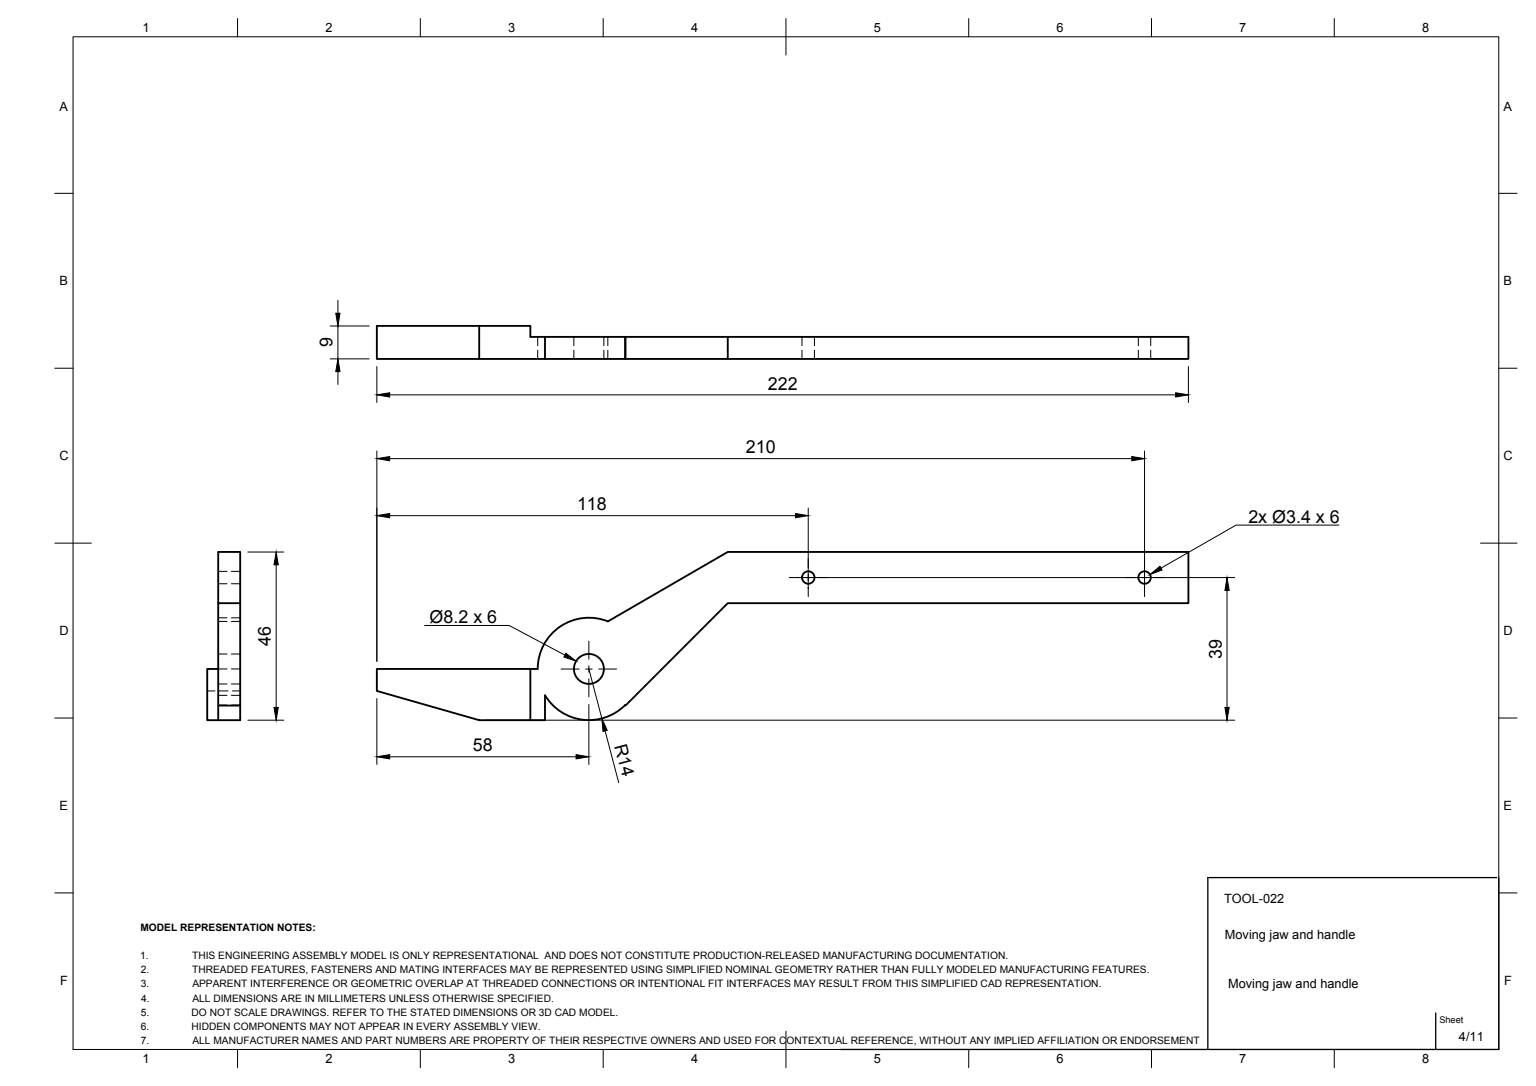
ISO-10303-21;
HEADER;
/* Generated by software containing ST-Developer
 * from STEP Tools, Inc. (www.steptools.com) 
 */

FILE_DESCRIPTION(
/* description */ (''),
/* implementation_level */ '2;1');

FILE_NAME(
/* name */ 'Moving jaw and handle.step',
/* time_stamp */ '2026-11-10T08:27:36-08:00',
/* author */ (''),
/* organization */ (''),
/* preprocessor_version */ 'ST-DEVELOPER v20.2',
/* originating_system */ 'Autodesk Translation Framework v15.17.0.0',
/* authorisation */ '');

FILE_SCHEMA (('AUTOMOTIVE_DESIGN { 1 0 10303 214 3 1 1 }'));
ENDSEC;

DATA;
#10=MECHANICAL_DESIGN_GEOMETRIC_PRESENTATION_REPRESENTATION('',(#567),#19090);
#547=SHAPE_REPRESENTATION_RELATIONSHIP('SRR','None',#19137,#557);
#557=ADVANCED_BREP_SHAPE_REPRESENTATION('',(#577),#19080);
#567=STYLED_ITEM('',(#19200),#577);
#577=MANIFOLD_SOLID_BREP('Body1',#6821);
#592=FACE_BOUND('',#1245,.T.);
#593=FACE_BOUND('',#1246,.T.);
#594=FACE_BOUND('',#1247,.T.);
#595=FACE_BOUND('',#1256,.T.);
#596=FACE_BOUND('',#1257,.T.);
#597=FACE_BOUND('',#1258,.T.);
#675=PLANE('',#6990);
#676=PLANE('',#6991);
#677=PLANE('',#6992);
#678=PLANE('',#6993);
#679=PLANE('',#6994);
#680=PLANE('',#6995);
#681=PLANE('',#6996);
#682=PLANE('',#6997);
#683=PLANE('',#7002);
#684=PLANE('',#7003);
#685=PLANE('',#7004);
#686=PLANE('',#7005);
#687=PLANE('',#7006);
#688=PLANE('',#7007);
#689=PLANE('',#7008);
#840=FACE_OUTER_BOUND('',#1234,.T.);
#841=FACE_OUTER_BOUND('',#1235,.T.);
#842=FACE_OUTER_BOUND('',#1236,.T.);
#843=FACE_OUTER_BOUND('',#1237,.T.);
#844=FACE_OUTER_BOUND('',#1238,.T.);
#845=FACE_OUTER_BOUND('',#1239,.T.);
#846=FACE_OUTER_BOUND('',#1240,.T.);
#847=FACE_OUTER_BOUND('',#1241,.T.);
#848=FACE_OUTER_BOUND('',#1242,.T.);
#849=FACE_OUTER_BOUND('',#1243,.T.);
#850=FACE_OUTER_BOUND('',#1244,.T.);
#851=FACE_OUTER_BOUND('',#1248,.T.);
#852=FACE_OUTER_BOUND('',#1249,.T.);
#853=FACE_OUTER_BOUND('',#1250,.T.);
#854=FACE_OUTER_BOUND('',#1251,.T.);
#855=FACE_OUTER_BOUND('',#1252,.T.);
#856=FACE_OUTER_BOUND('',#1253,.T.);
#857=FACE_OUTER_BOUND('',#1254,.T.);
#858=FACE_OUTER_BOUND('',#1255,.T.);
#859=FACE_OUTER_BOUND('',#1259,.T.);
#1234=EDGE_LOOP('',(#4477,#4478,#4479,#4480));
#1235=EDGE_LOOP('',(#4481,#4482,#4483,#4484));
#1236=EDGE_LOOP('',(#4485,#4486,#4487,#4488));
#1237=EDGE_LOOP('',(#4489,#4490,#4491,#4492));
#1238=EDGE_LOOP('',(#4493,#4494,#4495,#4496,#4497));
#1239=EDGE_LOOP('',(#4498,#4499,#4500,#4501,#4502,#4503));
#1240=EDGE_LOOP('',(#4504,#4505,#4506,#4507));
#1241=EDGE_LOOP('',(#4508,#4509,#4510,#4511));
#1242=EDGE_LOOP('',(#4512,#4513,#4514,#4515));
#1243=EDGE_LOOP('',(#4516,#4517,#4518,#4519,#4520,#4521));
#1244=EDGE_LOOP('',(#4522,#4523,#4524,#4525,#4526,#4527,#4528,#4529,#4530,
#4531,#4532,#4533));
#1245=EDGE_LOOP('',(#4534));
#1246=EDGE_LOOP('',(#4535));
#1247=EDGE_LOOP('',(#4536));
#1248=EDGE_LOOP('',(#4537,#4538,#4539,#4540));
#1249=EDGE_LOOP('',(#4541,#4542,#4543,#4544));
#1250=EDGE_LOOP('',(#4545,#4546,#4547,#4548));
#1251=EDGE_LOOP('',(#4549,#4550,#4551,#4552));
#1252=EDGE_LOOP('',(#4553,#4554,#4555,#4556));
#1253=EDGE_LOOP('',(#4557,#4558,#4559,#4560));
#1254=EDGE_LOOP('',(#4561,#4562,#4563,#4564));
#1255=EDGE_LOOP('',(#4565,#4566,#4567,#4568,#4569,#4570,#4571,#4572,#4573,
#4574,#4575,#4576,#4577));
#1256=EDGE_LOOP('',(#4578));
#1257=EDGE_LOOP('',(#4579));
#1258=EDGE_LOOP('',(#4580));
#1259=EDGE_LOOP('',(#4581,#4582,#4583,#4584));
#1717=LINE('',#9029,#2166);
#1718=LINE('',#9035,#2167);
#1719=LINE('',#9041,#2168);
#1720=LINE('',#9046,#2169);
#1721=LINE('',#9048,#2170);
#1722=LINE('',#9050,#2171);
#1723=LINE('',#9051,#2172);
#1724=LINE('',#9054,#2173);
#1725=LINE('',#9056,#2174);
#1726=LINE('',#9058,#2175);
#1727=LINE('',#9059,#2176);
#1728=LINE('',#9063,#2177);
#1729=LINE('',#9065,#2178);
#1730=LINE('',#9066,#2179);
#1731=LINE('',#9067,#2180);
#1732=LINE('',#9071,#2181);
#1733=LINE('',#9073,#2182);
#1734=LINE('',#9075,#2183);
#1735=LINE('',#9076,#2184);
#1736=LINE('',#9079,#2185);
#1737=LINE('',#9080,#2186);
#1738=LINE('',#9083,#2187);
#1739=LINE('',#9084,#2188);
#1740=LINE('',#9086,#2189);
#1741=LINE('',#9087,#2190);
#1742=LINE('',#9092,#2191);
#1743=LINE('',#9094,#2192);
#1744=LINE('',#9096,#2193);
#1745=LINE('',#9098,#2194);
#1746=LINE('',#9100,#2195);
#1747=LINE('',#9102,#2196);
#1748=LINE('',#9107,#2197);
#1749=LINE('',#9110,#2198);
#1750=LINE('',#9112,#2199);
#1751=LINE('',#9113,#2200);
#1752=LINE('',#9116,#2201);
#1753=LINE('',#9117,#2202);
#1754=LINE('',#9120,#2203);
#1755=LINE('',#9121,#2204);
#1756=LINE('',#9124,#2205);
#1757=LINE('',#9125,#2206);
#1758=LINE('',#9128,#2207);
#1759=LINE('',#9129,#2208);
#1760=LINE('',#9131,#2209);
#2166=VECTOR('',#7582,0.17);
#2167=VECTOR('',#7589,0.17);
#2168=VECTOR('',#7596,0.41);
#2169=VECTOR('',#7601,1.);
#2170=VECTOR('',#7602,1.);
#2171=VECTOR('',#7603,1.);
#2172=VECTOR('',#7604,1.);
#2173=VECTOR('',#7607,1.);
#2174=VECTOR('',#7608,1.);
#2175=VECTOR('',#7609,1.);
#2176=VECTOR('',#7610,1.);
#2177=VECTOR('',#7613,1.);
#2178=VECTOR('',#7614,1.);
#2179=VECTOR('',#7615,1.);
#2180=VECTOR('',#7616,1.);
#2181=VECTOR('',#7619,1.);
#2182=VECTOR('',#7620,1.);
#2183=VECTOR('',#7621,1.);
#2184=VECTOR('',#7622,1.);
#2185=VECTOR('',#7625,1.);
#2186=VECTOR('',#7626,1.);
#2187=VECTOR('',#7629,1.);
#2188=VECTOR('',#7630,1.);
#2189=VECTOR('',#7633,1.);
#2190=VECTOR('',#7634,1.);
#2191=VECTOR('',#7639,1.);
#2192=VECTOR('',#7640,1.);
#2193=VECTOR('',#7641,1.);
#2194=VECTOR('',#7642,1.);
#2195=VECTOR('',#7643,1.);
#2196=VECTOR('',#7644,1.);
#2197=VECTOR('',#7651,1.);
#2198=VECTOR('',#7654,1.);
#2199=VECTOR('',#7655,1.);
#2200=VECTOR('',#7656,1.);
#2201=VECTOR('',#7659,1.);
#2202=VECTOR('',#7660,1.);
#2203=VECTOR('',#7663,1.);
#2204=VECTOR('',#7664,1.);
#2205=VECTOR('',#7667,1.);
#2206=VECTOR('',#7668,1.);
#2207=VECTOR('',#7671,1.);
#2208=VECTOR('',#7672,1.);
#2209=VECTOR('',#7675,1.);
#2564=CIRCLE('',#6982,0.17);
#2565=CIRCLE('',#6983,0.17);
#2566=CIRCLE('',#6985,0.17);
#2567=CIRCLE('',#6986,0.17);
#2568=CIRCLE('',#6988,0.41);
#2569=CIRCLE('',#6989,0.41);
#2570=CIRCLE('',#6998,1.4);
#2571=CIRCLE('',#6999,1.4);
#2572=CIRCLE('',#7001,1.4);
#2573=CIRCLE('',#7009,1.4);
#2760=VERTEX_POINT('',#9026);
#2761=VERTEX_POINT('',#9028);
#2762=VERTEX_POINT('',#9032);
#2763=VERTEX_POINT('',#9034);
#2764=VERTEX_POINT('',#9038);
#2765=VERTEX_POINT('',#9040);
#2766=VERTEX_POINT('',#9044);
#2767=VERTEX_POINT('',#9045);
#2768=VERTEX_POINT('',#9047);
#2769=VERTEX_POINT('',#9049);
#2770=VERTEX_POINT('',#9053);
#2771=VERTEX_POINT('',#9055);
#2772=VERTEX_POINT('',#9057);
#2773=VERTEX_POINT('',#9061);
#2774=VERTEX_POINT('',#9062);
#2775=VERTEX_POINT('',#9064);
#2776=VERTEX_POINT('',#9069);
#2777=VERTEX_POINT('',#9070);
#2778=VERTEX_POINT('',#9072);
#2779=VERTEX_POINT('',#9074);
#2780=VERTEX_POINT('',#9078);
#2781=VERTEX_POINT('',#9082);
#2782=VERTEX_POINT('',#9089);
#2783=VERTEX_POINT('',#9091);
#2784=VERTEX_POINT('',#9093);
#2785=VERTEX_POINT('',#9095);
#2786=VERTEX_POINT('',#9097);
#2787=VERTEX_POINT('',#9099);
#2788=VERTEX_POINT('',#9101);
#2789=VERTEX_POINT('',#9105);
#2790=VERTEX_POINT('',#9109);
#2791=VERTEX_POINT('',#9111);
#2792=VERTEX_POINT('',#9115);
#2793=VERTEX_POINT('',#9119);
#2794=VERTEX_POINT('',#9123);
#2795=VERTEX_POINT('',#9127);
#3423=EDGE_CURVE('',#2760,#2760,#2564,.T.);
#3424=EDGE_CURVE('',#2760,#2761,#1717,.T.);
#3425=EDGE_CURVE('',#2761,#2761,#2565,.T.);
#3426=EDGE_CURVE('',#2762,#2762,#2566,.T.);
#3427=EDGE_CURVE('',#2762,#2763,#1718,.T.);
#3428=EDGE_CURVE('',#2763,#2763,#2567,.T.);
#3429=EDGE_CURVE('',#2764,#2764,#2568,.T.);
#3430=EDGE_CURVE('',#2764,#2765,#1719,.T.);
#3431=EDGE_CURVE('',#2765,#2765,#2569,.T.);
#3432=EDGE_CURVE('',#2766,#2767,#1720,.T.);
#3433=EDGE_CURVE('',#2766,#2768,#1721,.T.);
#3434=EDGE_CURVE('',#2769,#2768,#1722,.T.);
#3435=EDGE_CURVE('',#2767,#2769,#1723,.T.);
#3436=EDGE_CURVE('',#2770,#2766,#1724,.T.);
#3437=EDGE_CURVE('',#2767,#2771,#1725,.T.);
#3438=EDGE_CURVE('',#2771,#2772,#1726,.T.);
#3439=EDGE_CURVE('',#2772,#2770,#1727,.T.);
#3440=EDGE_CURVE('',#2773,#2774,#1728,.T.);
#3441=EDGE_CURVE('',#2775,#2773,#1729,.T.);
#3442=EDGE_CURVE('',#2771,#2775,#1730,.T.);
#3443=EDGE_CURVE('',#2774,#2769,#1731,.T.);
#3444=EDGE_CURVE('',#2776,#2777,#1732,.T.);
#3445=EDGE_CURVE('',#2778,#2776,#1733,.T.);
#3446=EDGE_CURVE('',#2778,#2779,#1734,.T.);
#3447=EDGE_CURVE('',#2777,#2779,#1735,.T.);
#3448=EDGE_CURVE('',#2780,#2775,#1736,.T.);
#3449=EDGE_CURVE('',#2772,#2780,#1737,.T.);
#3450=EDGE_CURVE('',#2781,#2780,#1738,.T.);
#3451=EDGE_CURVE('',#2770,#2781,#1739,.T.);
#3452=EDGE_CURVE('',#2779,#2781,#1740,.T.);
#3453=EDGE_CURVE('',#2768,#2778,#1741,.T.);
#3454=EDGE_CURVE('',#2782,#2776,#2570,.T.);
#3455=EDGE_CURVE('',#2783,#2782,#1742,.T.);
#3456=EDGE_CURVE('',#2784,#2783,#1743,.T.);
#3457=EDGE_CURVE('',#2785,#2784,#1744,.T.);
#3458=EDGE_CURVE('',#2786,#2785,#1745,.T.);
#3459=EDGE_CURVE('',#2787,#2786,#1746,.T.);
#3460=EDGE_CURVE('',#2788,#2787,#1747,.T.);
#3461=EDGE_CURVE('',#2774,#2788,#2571,.T.);
#3462=EDGE_CURVE('',#2789,#2777,#2572,.T.);
#3463=EDGE_CURVE('',#2789,#2782,#1748,.T.);
#3464=EDGE_CURVE('',#2788,#2790,#1749,.T.);
#3465=EDGE_CURVE('',#2787,#2791,#1750,.T.);
#3466=EDGE_CURVE('',#2790,#2791,#1751,.T.);
#3467=EDGE_CURVE('',#2792,#2789,#1752,.T.);
#3468=EDGE_CURVE('',#2783,#2792,#1753,.T.);
#3469=EDGE_CURVE('',#2793,#2792,#1754,.T.);
#3470=EDGE_CURVE('',#2784,#2793,#1755,.T.);
#3471=EDGE_CURVE('',#2794,#2793,#1756,.T.);
#3472=EDGE_CURVE('',#2785,#2794,#1757,.T.);
#3473=EDGE_CURVE('',#2795,#2794,#1758,.T.);
#3474=EDGE_CURVE('',#2786,#2795,#1759,.T.);
#3475=EDGE_CURVE('',#2791,#2795,#1760,.T.);
#3476=EDGE_CURVE('',#2773,#2790,#2573,.T.);
#4477=ORIENTED_EDGE('',*,*,#3423,.F.);
#4478=ORIENTED_EDGE('',*,*,#3424,.T.);
#4479=ORIENTED_EDGE('',*,*,#3425,.F.);
#4480=ORIENTED_EDGE('',*,*,#3424,.F.);
#4481=ORIENTED_EDGE('',*,*,#3426,.F.);
#4482=ORIENTED_EDGE('',*,*,#3427,.T.);
#4483=ORIENTED_EDGE('',*,*,#3428,.F.);
#4484=ORIENTED_EDGE('',*,*,#3427,.F.);
#4485=ORIENTED_EDGE('',*,*,#3429,.F.);
#4486=ORIENTED_EDGE('',*,*,#3430,.T.);
#4487=ORIENTED_EDGE('',*,*,#3431,.F.);
#4488=ORIENTED_EDGE('',*,*,#3430,.F.);
#4489=ORIENTED_EDGE('',*,*,#3432,.F.);
#4490=ORIENTED_EDGE('',*,*,#3433,.T.);
#4491=ORIENTED_EDGE('',*,*,#3434,.F.);
#4492=ORIENTED_EDGE('',*,*,#3435,.F.);
#4493=ORIENTED_EDGE('',*,*,#3436,.T.);
#4494=ORIENTED_EDGE('',*,*,#3432,.T.);
#4495=ORIENTED_EDGE('',*,*,#3437,.T.);
#4496=ORIENTED_EDGE('',*,*,#3438,.T.);
#4497=ORIENTED_EDGE('',*,*,#3439,.T.);
#4498=ORIENTED_EDGE('',*,*,#3440,.F.);
#4499=ORIENTED_EDGE('',*,*,#3441,.F.);
#4500=ORIENTED_EDGE('',*,*,#3442,.F.);
#4501=ORIENTED_EDGE('',*,*,#3437,.F.);
#4502=ORIENTED_EDGE('',*,*,#3435,.T.);
#4503=ORIENTED_EDGE('',*,*,#3443,.F.);
#4504=ORIENTED_EDGE('',*,*,#3444,.F.);
#4505=ORIENTED_EDGE('',*,*,#3445,.F.);
#4506=ORIENTED_EDGE('',*,*,#3446,.T.);
#4507=ORIENTED_EDGE('',*,*,#3447,.F.);
#4508=ORIENTED_EDGE('',*,*,#3442,.T.);
#4509=ORIENTED_EDGE('',*,*,#3448,.F.);
#4510=ORIENTED_EDGE('',*,*,#3449,.F.);
#4511=ORIENTED_EDGE('',*,*,#3438,.F.);
#4512=ORIENTED_EDGE('',*,*,#3449,.T.);
#4513=ORIENTED_EDGE('',*,*,#3450,.F.);
#4514=ORIENTED_EDGE('',*,*,#3451,.F.);
#4515=ORIENTED_EDGE('',*,*,#3439,.F.);
#4516=ORIENTED_EDGE('',*,*,#3451,.T.);
#4517=ORIENTED_EDGE('',*,*,#3452,.F.);
#4518=ORIENTED_EDGE('',*,*,#3446,.F.);
#4519=ORIENTED_EDGE('',*,*,#3453,.F.);
#4520=ORIENTED_EDGE('',*,*,#3433,.F.);
#4521=ORIENTED_EDGE('',*,*,#3436,.F.);
#4522=ORIENTED_EDGE('',*,*,#3434,.T.);
#4523=ORIENTED_EDGE('',*,*,#3453,.T.);
#4524=ORIENTED_EDGE('',*,*,#3445,.T.);
#4525=ORIENTED_EDGE('',*,*,#3454,.F.);
#4526=ORIENTED_EDGE('',*,*,#3455,.F.);
#4527=ORIENTED_EDGE('',*,*,#3456,.F.);
#4528=ORIENTED_EDGE('',*,*,#3457,.F.);
#4529=ORIENTED_EDGE('',*,*,#3458,.F.);
#4530=ORIENTED_EDGE('',*,*,#3459,.F.);
#4531=ORIENTED_EDGE('',*,*,#3460,.F.);
#4532=ORIENTED_EDGE('',*,*,#3461,.F.);
#4533=ORIENTED_EDGE('',*,*,#3443,.T.);
#4534=ORIENTED_EDGE('',*,*,#3425,.T.);
#4535=ORIENTED_EDGE('',*,*,#3428,.T.);
#4536=ORIENTED_EDGE('',*,*,#3431,.T.);
#4537=ORIENTED_EDGE('',*,*,#3444,.T.);
#4538=ORIENTED_EDGE('',*,*,#3462,.F.);
#4539=ORIENTED_EDGE('',*,*,#3463,.T.);
#4540=ORIENTED_EDGE('',*,*,#3454,.T.);
#4541=ORIENTED_EDGE('',*,*,#3464,.F.);
#4542=ORIENTED_EDGE('',*,*,#3460,.T.);
#4543=ORIENTED_EDGE('',*,*,#3465,.T.);
#4544=ORIENTED_EDGE('',*,*,#3466,.F.);
#4545=ORIENTED_EDGE('',*,*,#3463,.F.);
#4546=ORIENTED_EDGE('',*,*,#3467,.F.);
#4547=ORIENTED_EDGE('',*,*,#3468,.F.);
#4548=ORIENTED_EDGE('',*,*,#3455,.T.);
#4549=ORIENTED_EDGE('',*,*,#3456,.T.);
#4550=ORIENTED_EDGE('',*,*,#3468,.T.);
#4551=ORIENTED_EDGE('',*,*,#3469,.F.);
#4552=ORIENTED_EDGE('',*,*,#3470,.F.);
#4553=ORIENTED_EDGE('',*,*,#3457,.T.);
#4554=ORIENTED_EDGE('',*,*,#3470,.T.);
#4555=ORIENTED_EDGE('',*,*,#3471,.F.);
#4556=ORIENTED_EDGE('',*,*,#3472,.F.);
#4557=ORIENTED_EDGE('',*,*,#3458,.T.);
#4558=ORIENTED_EDGE('',*,*,#3472,.T.);
#4559=ORIENTED_EDGE('',*,*,#3473,.F.);
#4560=ORIENTED_EDGE('',*,*,#3474,.F.);
#4561=ORIENTED_EDGE('',*,*,#3459,.T.);
#4562=ORIENTED_EDGE('',*,*,#3474,.T.);
#4563=ORIENTED_EDGE('',*,*,#3475,.F.);
#4564=ORIENTED_EDGE('',*,*,#3465,.F.);
#4565=ORIENTED_EDGE('',*,*,#3476,.T.);
#4566=ORIENTED_EDGE('',*,*,#3466,.T.);
#4567=ORIENTED_EDGE('',*,*,#3475,.T.);
#4568=ORIENTED_EDGE('',*,*,#3473,.T.);
#4569=ORIENTED_EDGE('',*,*,#3471,.T.);
#4570=ORIENTED_EDGE('',*,*,#3469,.T.);
#4571=ORIENTED_EDGE('',*,*,#3467,.T.);
#4572=ORIENTED_EDGE('',*,*,#3462,.T.);
#4573=ORIENTED_EDGE('',*,*,#3447,.T.);
#4574=ORIENTED_EDGE('',*,*,#3452,.T.);
#4575=ORIENTED_EDGE('',*,*,#3450,.T.);
#4576=ORIENTED_EDGE('',*,*,#3448,.T.);
#4577=ORIENTED_EDGE('',*,*,#3441,.T.);
#4578=ORIENTED_EDGE('',*,*,#3423,.T.);
#4579=ORIENTED_EDGE('',*,*,#3426,.T.);
#4580=ORIENTED_EDGE('',*,*,#3429,.T.);
#4581=ORIENTED_EDGE('',*,*,#3440,.T.);
#4582=ORIENTED_EDGE('',*,*,#3461,.T.);
#4583=ORIENTED_EDGE('',*,*,#3464,.T.);
#4584=ORIENTED_EDGE('',*,*,#3476,.F.);
#6306=CYLINDRICAL_SURFACE('',#6981,0.17);
#6307=CYLINDRICAL_SURFACE('',#6984,0.17);
#6308=CYLINDRICAL_SURFACE('',#6987,0.41);
#6309=CYLINDRICAL_SURFACE('',#7000,1.4);
#6310=CYLINDRICAL_SURFACE('',#7010,1.4);
#6459=ADVANCED_FACE('',(#840),#6306,.F.);
#6460=ADVANCED_FACE('',(#841),#6307,.F.);
#6461=ADVANCED_FACE('',(#842),#6308,.F.);
#6462=ADVANCED_FACE('',(#843),#675,.T.);
#6463=ADVANCED_FACE('',(#844),#676,.F.);
#6464=ADVANCED_FACE('',(#845),#677,.T.);
#6465=ADVANCED_FACE('',(#846),#678,.T.);
#6466=ADVANCED_FACE('',(#847),#679,.T.);
#6467=ADVANCED_FACE('',(#848),#680,.T.);
#6468=ADVANCED_FACE('',(#849),#681,.T.);
#6469=ADVANCED_FACE('',(#850,#592,#593,#594),#682,.F.);
#6470=ADVANCED_FACE('',(#851),#6309,.T.);
#6471=ADVANCED_FACE('',(#852),#683,.T.);
#6472=ADVANCED_FACE('',(#853),#684,.T.);
#6473=ADVANCED_FACE('',(#854),#685,.T.);
#6474=ADVANCED_FACE('',(#855),#686,.T.);
#6475=ADVANCED_FACE('',(#856),#687,.T.);
#6476=ADVANCED_FACE('',(#857),#688,.T.);
#6477=ADVANCED_FACE('',(#858,#595,#596,#597),#689,.T.);
#6478=ADVANCED_FACE('',(#859),#6310,.T.);
#6821=CLOSED_SHELL('',(#6459,#6460,#6461,#6462,#6463,#6464,#6465,#6466,
#6467,#6468,#6469,#6470,#6471,#6472,#6473,#6474,#6475,#6476,#6477,#6478));
#6980=AXIS2_PLACEMENT_3D('',#9024,#7576,#7577);
#6981=AXIS2_PLACEMENT_3D('',#9025,#7578,#7579);
#6982=AXIS2_PLACEMENT_3D('',#9027,#7580,#7581);
#6983=AXIS2_PLACEMENT_3D('',#9030,#7583,#7584);
#6984=AXIS2_PLACEMENT_3D('',#9031,#7585,#7586);
#6985=AXIS2_PLACEMENT_3D('',#9033,#7587,#7588);
#6986=AXIS2_PLACEMENT_3D('',#9036,#7590,#7591);
#6987=AXIS2_PLACEMENT_3D('',#9037,#7592,#7593);
#6988=AXIS2_PLACEMENT_3D('',#9039,#7594,#7595);
#6989=AXIS2_PLACEMENT_3D('',#9042,#7597,#7598);
#6990=AXIS2_PLACEMENT_3D('',#9043,#7599,#7600);
#6991=AXIS2_PLACEMENT_3D('',#9052,#7605,#7606);
#6992=AXIS2_PLACEMENT_3D('',#9060,#7611,#7612);
#6993=AXIS2_PLACEMENT_3D('',#9068,#7617,#7618);
#6994=AXIS2_PLACEMENT_3D('',#9077,#7623,#7624);
#6995=AXIS2_PLACEMENT_3D('',#9081,#7627,#7628);
#6996=AXIS2_PLACEMENT_3D('',#9085,#7631,#7632);
#6997=AXIS2_PLACEMENT_3D('',#9088,#7635,#7636);
#6998=AXIS2_PLACEMENT_3D('',#9090,#7637,#7638);
#6999=AXIS2_PLACEMENT_3D('',#9103,#7645,#7646);
#7000=AXIS2_PLACEMENT_3D('',#9104,#7647,#7648);
#7001=AXIS2_PLACEMENT_3D('',#9106,#7649,#7650);
#7002=AXIS2_PLACEMENT_3D('',#9108,#7652,#7653);
#7003=AXIS2_PLACEMENT_3D('',#9114,#7657,#7658);
#7004=AXIS2_PLACEMENT_3D('',#9118,#7661,#7662);
#7005=AXIS2_PLACEMENT_3D('',#9122,#7665,#7666);
#7006=AXIS2_PLACEMENT_3D('',#9126,#7669,#7670);
#7007=AXIS2_PLACEMENT_3D('',#9130,#7673,#7674);
#7008=AXIS2_PLACEMENT_3D('',#9132,#7676,#7677);
#7009=AXIS2_PLACEMENT_3D('',#9133,#7678,#7679);
#7010=AXIS2_PLACEMENT_3D('',#9134,#7680,#7681);
#7576=DIRECTION('axis',(0.,0.,1.));
#7577=DIRECTION('refdir',(1.,0.,0.));
#7578=DIRECTION('center_axis',(0.,0.,-1.));
#7579=DIRECTION('ref_axis',(1.,0.,0.));
#7580=DIRECTION('center_axis',(0.,0.,-1.));
#7581=DIRECTION('ref_axis',(1.,0.,0.));
#7582=DIRECTION('',(0.,0.,-1.));
#7583=DIRECTION('center_axis',(0.,0.,1.));
#7584=DIRECTION('ref_axis',(1.,0.,0.));
#7585=DIRECTION('center_axis',(0.,0.,-1.));
#7586=DIRECTION('ref_axis',(1.,0.,0.));
#7587=DIRECTION('center_axis',(0.,0.,-1.));
#7588=DIRECTION('ref_axis',(1.,0.,0.));
#7589=DIRECTION('',(0.,0.,-1.));
#7590=DIRECTION('center_axis',(0.,0.,1.));
#7591=DIRECTION('ref_axis',(1.,0.,0.));
#7592=DIRECTION('center_axis',(0.,0.,-1.));
#7593=DIRECTION('ref_axis',(1.,0.,0.));
#7594=DIRECTION('center_axis',(0.,0.,-1.));
#7595=DIRECTION('ref_axis',(1.,0.,0.));
#7596=DIRECTION('',(0.,0.,-1.));
#7597=DIRECTION('center_axis',(0.,0.,1.));
#7598=DIRECTION('ref_axis',(1.,0.,0.));
#7599=DIRECTION('center_axis',(1.,0.,0.));
#7600=DIRECTION('ref_axis',(0.,1.,0.));
#7601=DIRECTION('',(0.,-1.,0.));
#7602=DIRECTION('',(0.,0.,1.));
#7603=DIRECTION('',(0.,1.,0.));
#7604=DIRECTION('',(0.,0.,1.));
#7605=DIRECTION('center_axis',(0.,0.,1.));
#7606=DIRECTION('ref_axis',(1.,0.,0.));
#7607=DIRECTION('',(1.,0.,0.));
#7608=DIRECTION('',(-1.,0.,0.));
#7609=DIRECTION('',(0.,1.,0.));
#7610=DIRECTION('',(0.961523947640823,0.274721127897378,0.));
#7611=DIRECTION('center_axis',(0.,-1.,0.));
#7612=DIRECTION('ref_axis',(1.,0.,0.));
#7613=DIRECTION('',(0.,0.,-1.));
#7614=DIRECTION('',(1.,0.,0.));
#7615=DIRECTION('',(0.,0.,1.));
#7616=DIRECTION('',(-1.,0.,0.));
#7617=DIRECTION('center_axis',(1.,0.,0.));
#7618=DIRECTION('ref_axis',(0.,1.,0.));
#7619=DIRECTION('',(0.,0.,1.));
#7620=DIRECTION('',(0.,-1.,0.));
#7621=DIRECTION('',(0.,0.,1.));
#7622=DIRECTION('',(0.,1.,0.));
#7623=DIRECTION('center_axis',(-1.,0.,0.));
#7624=DIRECTION('ref_axis',(0.,-1.,0.));
#7625=DIRECTION('',(0.,-1.,0.));
#7626=DIRECTION('',(0.,0.,1.));
#7627=DIRECTION('center_axis',(-0.274721127897378,0.961523947640823,0.));
#7628=DIRECTION('ref_axis',(-0.961523947640823,-0.274721127897378,0.));
#7629=DIRECTION('',(-0.961523947640823,-0.274721127897378,0.));
#7630=DIRECTION('',(0.,0.,1.));
#7631=DIRECTION('center_axis',(0.,1.,0.));
#7632=DIRECTION('ref_axis',(-1.,0.,0.));
#7633=DIRECTION('',(-1.,0.,0.));
#7634=DIRECTION('',(1.,0.,0.));
#7635=DIRECTION('center_axis',(0.,0.,1.));
#7636=DIRECTION('ref_axis',(1.,0.,0.));
#7637=DIRECTION('center_axis',(0.,0.,1.));
#7638=DIRECTION('ref_axis',(1.,0.,0.));
#7639=DIRECTION('',(-0.447213595499958,-0.894427190999916,0.));
#7640=DIRECTION('',(-0.707106781186548,0.707106781186548,0.));
#7641=DIRECTION('',(-1.,0.,0.));
#7642=DIRECTION('',(0.,1.,0.));
#7643=DIRECTION('',(1.,0.,0.));
#7644=DIRECTION('',(0.865426285481126,-0.501036270541705,0.));
#7645=DIRECTION('center_axis',(0.,0.,1.));
#7646=DIRECTION('ref_axis',(1.,0.,0.));
#7647=DIRECTION('center_axis',(0.,0.,1.));
#7648=DIRECTION('ref_axis',(1.,0.,0.));
#7649=DIRECTION('center_axis',(0.,0.,1.));
#7650=DIRECTION('ref_axis',(1.,0.,0.));
#7651=DIRECTION('',(0.,0.,-1.));
#7652=DIRECTION('center_axis',(-0.501036270541705,-0.865426285481126,0.));
#7653=DIRECTION('ref_axis',(0.865426285481126,-0.501036270541705,0.));
#7654=DIRECTION('',(0.,0.,1.));
#7655=DIRECTION('',(0.,0.,1.));
#7656=DIRECTION('',(0.865426285481126,-0.501036270541705,0.));
#7657=DIRECTION('center_axis',(-0.894427190999916,0.447213595499958,0.));
#7658=DIRECTION('ref_axis',(-0.447213595499958,-0.894427190999916,0.));
#7659=DIRECTION('',(-0.447213595499958,-0.894427190999916,0.));
#7660=DIRECTION('',(0.,0.,1.));
#7661=DIRECTION('center_axis',(0.707106781186548,0.707106781186548,0.));
#7662=DIRECTION('ref_axis',(-0.707106781186548,0.707106781186548,0.));
#7663=DIRECTION('',(-0.707106781186548,0.707106781186548,0.));
#7664=DIRECTION('',(0.,0.,1.));
#7665=DIRECTION('center_axis',(0.,1.,0.));
#7666=DIRECTION('ref_axis',(-1.,0.,0.));
#7667=DIRECTION('',(-1.,0.,0.));
#7668=DIRECTION('',(0.,0.,1.));
#7669=DIRECTION('center_axis',(1.,0.,0.));
#7670=DIRECTION('ref_axis',(0.,1.,0.));
#7671=DIRECTION('',(0.,1.,0.));
#7672=DIRECTION('',(0.,0.,1.));
#7673=DIRECTION('center_axis',(0.,-1.,0.));
#7674=DIRECTION('ref_axis',(1.,0.,0.));
#7675=DIRECTION('',(1.,0.,0.));
#7676=DIRECTION('center_axis',(0.,0.,1.));
#7677=DIRECTION('ref_axis',(1.,0.,0.));
#7678=DIRECTION('center_axis',(0.,0.,1.));
#7679=DIRECTION('ref_axis',(1.,0.,0.));
#7680=DIRECTION('center_axis',(0.,0.,1.));
#7681=DIRECTION('ref_axis',(1.,0.,0.));
#9024=CARTESIAN_POINT('',(0.,0.,0.));
#9025=CARTESIAN_POINT('Origin',(6.,-2.5,0.3));
#9026=CARTESIAN_POINT('',(5.83,-2.5,0.6));
#9027=CARTESIAN_POINT('Origin',(6.,-2.5,0.6));
#9028=CARTESIAN_POINT('',(5.83,-2.5,0.));
#9029=CARTESIAN_POINT('',(5.83,-2.5,0.3));
#9030=CARTESIAN_POINT('Origin',(6.,-2.5,0.));
#9031=CARTESIAN_POINT('Origin',(15.2,-2.5,0.3));
#9032=CARTESIAN_POINT('',(15.03,-2.5,0.6));
#9033=CARTESIAN_POINT('Origin',(15.2,-2.5,0.6));
#9034=CARTESIAN_POINT('',(15.03,-2.5,0.));
#9035=CARTESIAN_POINT('',(15.03,-2.5,0.3));
#9036=CARTESIAN_POINT('Origin',(15.2,-2.5,0.));
#9037=CARTESIAN_POINT('Origin',(0.,0.,0.3));
#9038=CARTESIAN_POINT('',(-0.41,5.02105187650415E-17,0.6));
#9039=CARTESIAN_POINT('Origin',(0.,0.,0.6));
#9040=CARTESIAN_POINT('',(-0.41,5.02105187650415E-17,0.));
#9041=CARTESIAN_POINT('',(-0.41,5.02105187650415E-17,0.3));
#9042=CARTESIAN_POINT('Origin',(0.,0.,0.));
#9043=CARTESIAN_POINT('Origin',(-1.6,0.,-0.3));
#9044=CARTESIAN_POINT('',(-1.6,1.4,-0.3));
#9045=CARTESIAN_POINT('',(-1.6,0.,-0.3));
#9046=CARTESIAN_POINT('',(-1.6,1.4,-0.3));
#9047=CARTESIAN_POINT('',(-1.6,1.4,0.));
#9048=CARTESIAN_POINT('',(-1.6,1.4,-0.3));
#9049=CARTESIAN_POINT('',(-1.6,0.,0.));
#9050=CARTESIAN_POINT('',(-1.6,0.,0.));
#9051=CARTESIAN_POINT('',(-1.6,0.,-0.3));
#9052=CARTESIAN_POINT('Origin',(-3.7,0.7,-0.3));
#9053=CARTESIAN_POINT('',(-3.,1.4,-0.3));
#9054=CARTESIAN_POINT('',(-3.,1.4,-0.3));
#9055=CARTESIAN_POINT('',(-5.8,0.,-0.3));
#9056=CARTESIAN_POINT('',(-1.6,0.,-0.3));
#9057=CARTESIAN_POINT('',(-5.8,0.6,-0.3));
#9058=CARTESIAN_POINT('',(-5.8,0.,-0.3));
#9059=CARTESIAN_POINT('',(-5.8,0.6,-0.3));
#9060=CARTESIAN_POINT('Origin',(-5.8,0.,0.));
#9061=CARTESIAN_POINT('',(-1.4,0.,0.6));
#9062=CARTESIAN_POINT('',(-1.4,0.,0.));
#9063=CARTESIAN_POINT('',(-1.4,0.,0.));
#9064=CARTESIAN_POINT('',(-5.8,0.,0.6));
#9065=CARTESIAN_POINT('',(-1.2,0.,0.6));
#9066=CARTESIAN_POINT('',(-5.8,0.,0.));
#9067=CARTESIAN_POINT('',(-1.2,0.,0.));
#9068=CARTESIAN_POINT('Origin',(-1.2,0.,0.));
#9069=CARTESIAN_POINT('',(-1.2,0.721110255092798,0.));
#9070=CARTESIAN_POINT('',(-1.2,0.721110255092798,0.6));
#9071=CARTESIAN_POINT('',(-1.2,0.721110255092798,0.));
#9072=CARTESIAN_POINT('',(-1.2,1.4,0.));
#9073=CARTESIAN_POINT('',(-1.2,1.4,0.));
#9074=CARTESIAN_POINT('',(-1.2,1.4,0.6));
#9075=CARTESIAN_POINT('',(-1.2,1.4,0.));
#9076=CARTESIAN_POINT('',(-1.2,1.4,0.6));
#9077=CARTESIAN_POINT('Origin',(-5.8,0.6,0.));
#9078=CARTESIAN_POINT('',(-5.8,0.6,0.6));
#9079=CARTESIAN_POINT('',(-5.8,0.,0.6));
#9080=CARTESIAN_POINT('',(-5.8,0.6,0.));
#9081=CARTESIAN_POINT('Origin',(-3.,1.4,0.));
#9082=CARTESIAN_POINT('',(-3.,1.4,0.6));
#9083=CARTESIAN_POINT('',(-5.8,0.6,0.6));
#9084=CARTESIAN_POINT('',(-3.,1.4,0.));
#9085=CARTESIAN_POINT('Origin',(-1.2,1.4,0.));
#9086=CARTESIAN_POINT('',(-3.,1.4,0.6));
#9087=CARTESIAN_POINT('',(-3.,1.4,0.));
#9088=CARTESIAN_POINT('Origin',(0.,0.,0.));
#9089=CARTESIAN_POINT('',(0.993295878967653,0.986591757935306,0.));
#9090=CARTESIAN_POINT('Origin',(0.,0.,0.));
#9091=CARTESIAN_POINT('',(1.,1.,0.));
#9092=CARTESIAN_POINT('',(1.,1.,0.));
#9093=CARTESIAN_POINT('',(3.8,-1.8,0.));
#9094=CARTESIAN_POINT('',(3.8,-1.8,0.));
#9095=CARTESIAN_POINT('',(16.4,-1.8,0.));
#9096=CARTESIAN_POINT('',(16.4,-1.8,0.));
#9097=CARTESIAN_POINT('',(16.4,-3.2,0.));
#9098=CARTESIAN_POINT('',(16.4,-3.2,0.));
#9099=CARTESIAN_POINT('',(3.8,-3.2,0.));
#9100=CARTESIAN_POINT('',(3.8,-3.2,0.));
#9101=CARTESIAN_POINT('',(0.518766934059614,-1.30033875129767,0.));
#9102=CARTESIAN_POINT('',(0.,-1.,0.));
#9103=CARTESIAN_POINT('Origin',(0.,0.,0.));
#9104=CARTESIAN_POINT('Origin',(0.,0.,0.));
#9105=CARTESIAN_POINT('',(0.993295878967653,0.986591757935306,0.6));
#9106=CARTESIAN_POINT('Origin',(0.,0.,0.6));
#9107=CARTESIAN_POINT('',(0.993295878967653,0.986591757935306,0.));
#9108=CARTESIAN_POINT('Origin',(0.,-1.,0.));
#9109=CARTESIAN_POINT('',(0.518766934059614,-1.30033875129767,0.6));
#9110=CARTESIAN_POINT('',(0.518766934059614,-1.30033875129767,0.));
#9111=CARTESIAN_POINT('',(3.8,-3.2,0.6));
#9112=CARTESIAN_POINT('',(3.8,-3.2,0.));
#9113=CARTESIAN_POINT('',(0.,-1.,0.6));
#9114=CARTESIAN_POINT('Origin',(1.,1.,0.));
#9115=CARTESIAN_POINT('',(1.,1.,0.6));
#9116=CARTESIAN_POINT('',(1.,1.,0.6));
#9117=CARTESIAN_POINT('',(1.,1.,0.));
#9118=CARTESIAN_POINT('Origin',(3.8,-1.8,0.));
#9119=CARTESIAN_POINT('',(3.8,-1.8,0.6));
#9120=CARTESIAN_POINT('',(3.8,-1.8,0.6));
#9121=CARTESIAN_POINT('',(3.8,-1.8,0.));
#9122=CARTESIAN_POINT('Origin',(16.4,-1.8,0.));
#9123=CARTESIAN_POINT('',(16.4,-1.8,0.6));
#9124=CARTESIAN_POINT('',(16.4,-1.8,0.6));
#9125=CARTESIAN_POINT('',(16.4,-1.8,0.));
#9126=CARTESIAN_POINT('Origin',(16.4,-3.2,0.));
#9127=CARTESIAN_POINT('',(16.4,-3.2,0.6));
#9128=CARTESIAN_POINT('',(16.4,-3.2,0.6));
#9129=CARTESIAN_POINT('',(16.4,-3.2,0.));
#9130=CARTESIAN_POINT('Origin',(3.8,-3.2,0.));
#9131=CARTESIAN_POINT('',(3.8,-3.2,0.6));
#9132=CARTESIAN_POINT('Origin',(0.,0.,0.6));
#9133=CARTESIAN_POINT('Origin',(0.,0.,0.6));
#9134=CARTESIAN_POINT('Origin',(0.,0.,0.));
#19067=UNCERTAINTY_MEASURE_WITH_UNIT(LENGTH_MEASURE(0.001),#19091,
'DISTANCE_ACCURACY_VALUE',
'Maximum model space distance between geometric entities at asserted c
onnectivities');
#19077=UNCERTAINTY_MEASURE_WITH_UNIT(LENGTH_MEASURE(0.001),#19091,
'DISTANCE_ACCURACY_VALUE',
'Maximum model space distance between geometric entities at asserted c
onnectivities');
#19080=(
GEOMETRIC_REPRESENTATION_CONTEXT(3)
GLOBAL_UNCERTAINTY_ASSIGNED_CONTEXT((#19067))
GLOBAL_UNIT_ASSIGNED_CONTEXT((#19091,#19093,#19094))
REPRESENTATION_CONTEXT('','3D')
);
#19090=(
GEOMETRIC_REPRESENTATION_CONTEXT(3)
GLOBAL_UNCERTAINTY_ASSIGNED_CONTEXT((#19077))
GLOBAL_UNIT_ASSIGNED_CONTEXT((#19091,#19093,#19094))
REPRESENTATION_CONTEXT('','3D')
);
#19091=(
LENGTH_UNIT()
NAMED_UNIT(*)
SI_UNIT(.CENTI.,.METRE.)
);
#19093=(
NAMED_UNIT(*)
PLANE_ANGLE_UNIT()
SI_UNIT($,.RADIAN.)
);
#19094=(
NAMED_UNIT(*)
SI_UNIT($,.STERADIAN.)
SOLID_ANGLE_UNIT()
);
#19097=SHAPE_DEFINITION_REPRESENTATION(#19109,#19137);
#19109=PRODUCT_DEFINITION_SHAPE('',$,#19150);
#19137=SHAPE_REPRESENTATION('',(#6980),#19080);
#19147=PRODUCT_DEFINITION_CONTEXT('part definition',#19185,'design');
#19150=PRODUCT_DEFINITION('Moving jaw and handle',
'Moving jaw and handle',#19162,#19147);
#19162=PRODUCT_DEFINITION_FORMATION('',$,#19189);
#19185=APPLICATION_CONTEXT(
'Core Data for Automotive Mechanical Design Process');
#19186=PRODUCT_CONTEXT('part definition',#19185,'mechanical');
#19189=PRODUCT('Moving jaw and handle','Moving jaw and handle',$,(#19186));
#19200=PRESENTATION_STYLE_ASSIGNMENT((#19208));
#19208=SURFACE_STYLE_USAGE(.BOTH.,#19216);
#19216=SURFACE_SIDE_STYLE('',(#19224));
#19224=SURFACE_STYLE_FILL_AREA(#19232);
#19232=FILL_AREA_STYLE('Tool steel gray',(#19240));
#19240=FILL_AREA_STYLE_COLOUR('Tool steel gray',#19248);
#19248=COLOUR_RGB('Tool steel gray',0.607843137254902,0.643137254901961,
0.698039215686274);
ENDSEC;
END-ISO-10303-21;
